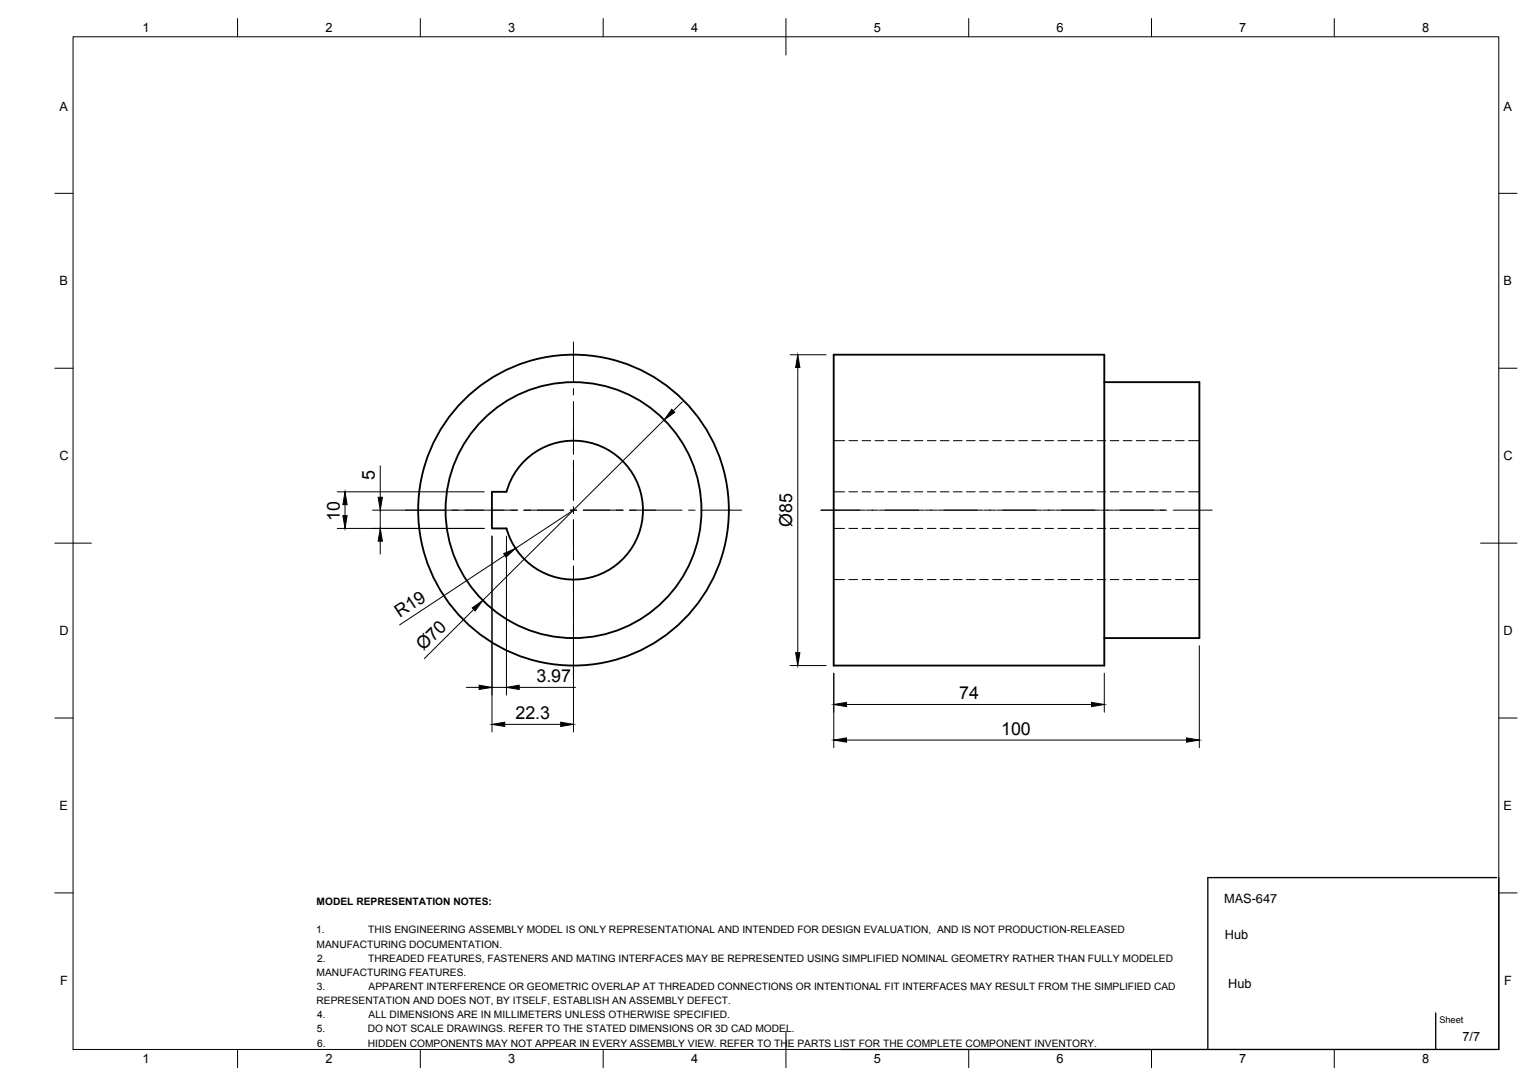
ISO-10303-21;
HEADER;
FILE_DESCRIPTION((''),'2;1');
FILE_NAME('Hub.step','2026-10-09T11:36:02-07:00',(''),(''),'','','');
FILE_SCHEMA (('AUTOMOTIVE_DESIGN { 1 0 10303 214 3 1 1 }'));
ENDSEC;
DATA;
#10=MECHANICAL_DESIGN_GEOMETRIC_PRESENTATION_REPRESENTATION('',(#85),#1549);
#75=SHAPE_REPRESENTATION_RELATIONSHIP('SRR','None',#1584,#80) ;
#80=ADVANCED_BREP_SHAPE_REPRESENTATION('',(#90),#1547) ;
#85=STYLED_ITEM('',(#1615),#90) ;
#90=MANIFOLD_SOLID_BREP('Body1',#847) ;
#120=FACE_BOUND('',#246,.T.) ;
#121=FACE_BOUND('',#248,.T.) ;
#122=FACE_BOUND('',#250,.T.) ;
#127=PLANE('',#988) ;
#128=PLANE('',#989) ;
#129=PLANE('',#990) ;
#130=PLANE('',#991) ;
#131=PLANE('',#992) ;
#132=PLANE('',#993) ;
#168=FACE_OUTER_BOUND('',#242,.T.) ;
#169=FACE_OUTER_BOUND('',#243,.T.) ;
#170=FACE_OUTER_BOUND('',#244,.T.) ;
#171=FACE_OUTER_BOUND('',#245,.T.) ;
#172=FACE_OUTER_BOUND('',#247,.T.) ;
#173=FACE_OUTER_BOUND('',#249,.T.) ;
#174=FACE_OUTER_BOUND('',#251,.T.) ;
#175=FACE_OUTER_BOUND('',#252,.T.) ;
#176=FACE_OUTER_BOUND('',#253,.T.) ;
#242=EDGE_LOOP('',(#699,#700,#701,#702)) ;
#243=EDGE_LOOP('',(#703,#704,#705,#706)) ;
#244=EDGE_LOOP('',(#707,#708,#709,#710)) ;
#245=EDGE_LOOP('',(#711)) ;
#246=EDGE_LOOP('',(#712,#713,#714,#715)) ;
#247=EDGE_LOOP('',(#716)) ;
#248=EDGE_LOOP('',(#717)) ;
#249=EDGE_LOOP('',(#718)) ;
#250=EDGE_LOOP('',(#719,#720,#721,#722)) ;
#251=EDGE_LOOP('',(#723,#724,#725,#726)) ;
#252=EDGE_LOOP('',(#727,#728,#729,#730)) ;
#253=EDGE_LOOP('',(#731,#732,#733,#734)) ;
#284=LINE('',#1444,#332) ;
#285=LINE('',#1450,#333) ;
#286=LINE('',#1457,#334) ;
#287=LINE('',#1460,#335) ;
#288=LINE('',#1464,#336) ;
#289=LINE('',#1465,#337) ;
#290=LINE('',#1466,#338) ;
#291=LINE('',#1470,#339) ;
#292=LINE('',#1472,#340) ;
#293=LINE('',#1473,#341) ;
#294=LINE('',#1475,#342) ;
#295=LINE('',#1477,#343) ;
#332=VECTOR('',#1195,42.5) ;
#333=VECTOR('',#1202,35.) ;
#334=VECTOR('',#1209,1000.) ;
#335=VECTOR('',#1212,1000.) ;
#336=VECTOR('',#1215,1000.) ;
#337=VECTOR('',#1216,1000.) ;
#338=VECTOR('',#1217,1000.) ;
#339=VECTOR('',#1222,1000.) ;
#340=VECTOR('',#1223,1000.) ;
#341=VECTOR('',#1224,1000.) ;
#342=VECTOR('',#1227,1000.) ;
#343=VECTOR('',#1230,1000.) ;
#402=CIRCLE('',#980,42.5) ;
#403=CIRCLE('',#981,42.5) ;
#404=CIRCLE('',#983,35.) ;
#405=CIRCLE('',#984,35.) ;
#406=CIRCLE('',#986,19.) ;
#407=CIRCLE('',#987,19.) ;
#451=VERTEX_POINT('',#1441) ;
#452=VERTEX_POINT('',#1443) ;
#453=VERTEX_POINT('',#1447) ;
#454=VERTEX_POINT('',#1449) ;
#455=VERTEX_POINT('',#1453) ;
#456=VERTEX_POINT('',#1454) ;
#457=VERTEX_POINT('',#1456) ;
#458=VERTEX_POINT('',#1458) ;
#459=VERTEX_POINT('',#1462) ;
#460=VERTEX_POINT('',#1463) ;
#461=VERTEX_POINT('',#1469) ;
#462=VERTEX_POINT('',#1471) ;
#537=EDGE_CURVE('',#451,#451,#402,.T.) ;
#538=EDGE_CURVE('',#451,#452,#284,.T.) ;
#539=EDGE_CURVE('',#452,#452,#403,.T.) ;
#540=EDGE_CURVE('',#453,#453,#404,.T.) ;
#541=EDGE_CURVE('',#453,#454,#285,.T.) ;
#542=EDGE_CURVE('',#454,#454,#405,.T.) ;
#543=EDGE_CURVE('',#455,#456,#406,.T.) ;
#544=EDGE_CURVE('',#457,#455,#286,.T.) ;
#545=EDGE_CURVE('',#457,#458,#407,.T.) ;
#546=EDGE_CURVE('',#458,#456,#287,.T.) ;
#547=EDGE_CURVE('',#459,#460,#288,.T.) ;
#548=EDGE_CURVE('',#460,#458,#289,.T.) ;
#549=EDGE_CURVE('',#457,#459,#290,.T.) ;
#550=EDGE_CURVE('',#461,#456,#291,.T.) ;
#551=EDGE_CURVE('',#462,#461,#292,.T.) ;
#552=EDGE_CURVE('',#455,#462,#293,.T.) ;
#553=EDGE_CURVE('',#460,#461,#294,.T.) ;
#554=EDGE_CURVE('',#459,#462,#295,.T.) ;
#699=ORIENTED_EDGE('',*,*,#537,.F.) ;
#700=ORIENTED_EDGE('',*,*,#538,.T.) ;
#701=ORIENTED_EDGE('',*,*,#539,.T.) ;
#702=ORIENTED_EDGE('',*,*,#538,.F.) ;
#703=ORIENTED_EDGE('',*,*,#540,.F.) ;
#704=ORIENTED_EDGE('',*,*,#541,.T.) ;
#705=ORIENTED_EDGE('',*,*,#542,.T.) ;
#706=ORIENTED_EDGE('',*,*,#541,.F.) ;
#707=ORIENTED_EDGE('',*,*,#543,.F.) ;
#708=ORIENTED_EDGE('',*,*,#544,.F.) ;
#709=ORIENTED_EDGE('',*,*,#545,.T.) ;
#710=ORIENTED_EDGE('',*,*,#546,.T.) ;
#711=ORIENTED_EDGE('',*,*,#540,.T.) ;
#712=ORIENTED_EDGE('',*,*,#547,.T.) ;
#713=ORIENTED_EDGE('',*,*,#548,.T.) ;
#714=ORIENTED_EDGE('',*,*,#545,.F.) ;
#715=ORIENTED_EDGE('',*,*,#549,.T.) ;
#716=ORIENTED_EDGE('',*,*,#537,.T.) ;
#717=ORIENTED_EDGE('',*,*,#542,.F.) ;
#718=ORIENTED_EDGE('',*,*,#539,.F.) ;
#719=ORIENTED_EDGE('',*,*,#543,.T.) ;
#720=ORIENTED_EDGE('',*,*,#550,.F.) ;
#721=ORIENTED_EDGE('',*,*,#551,.F.) ;
#722=ORIENTED_EDGE('',*,*,#552,.F.) ;
#723=ORIENTED_EDGE('',*,*,#550,.T.) ;
#724=ORIENTED_EDGE('',*,*,#546,.F.) ;
#725=ORIENTED_EDGE('',*,*,#548,.F.) ;
#726=ORIENTED_EDGE('',*,*,#553,.T.) ;
#727=ORIENTED_EDGE('',*,*,#551,.T.) ;
#728=ORIENTED_EDGE('',*,*,#553,.F.) ;
#729=ORIENTED_EDGE('',*,*,#547,.F.) ;
#730=ORIENTED_EDGE('',*,*,#554,.T.) ;
#731=ORIENTED_EDGE('',*,*,#552,.T.) ;
#732=ORIENTED_EDGE('',*,*,#554,.F.) ;
#733=ORIENTED_EDGE('',*,*,#549,.F.) ;
#734=ORIENTED_EDGE('',*,*,#544,.T.) ;
#793=CYLINDRICAL_SURFACE('',#979,42.5) ;
#794=CYLINDRICAL_SURFACE('',#982,35.) ;
#795=CYLINDRICAL_SURFACE('',#985,19.) ;
#825=ADVANCED_FACE('',(#168),#793,.T.) ;
#826=ADVANCED_FACE('',(#169),#794,.T.) ;
#827=ADVANCED_FACE('',(#170),#795,.F.) ;
#828=ADVANCED_FACE('',(#171,#120),#127,.F.) ;
#829=ADVANCED_FACE('',(#172,#121),#128,.F.) ;
#830=ADVANCED_FACE('',(#173,#122),#129,.F.) ;
#831=ADVANCED_FACE('',(#174),#130,.F.) ;
#832=ADVANCED_FACE('',(#175),#131,.F.) ;
#833=ADVANCED_FACE('',(#176),#132,.F.) ;
#847=CLOSED_SHELL('',(#825,#826,#827,#828,#829,#830,#831,#832,#833)) ;
#978=AXIS2_PLACEMENT_3D('',#1439,#1189,#1190) ;
#979=AXIS2_PLACEMENT_3D('',#1440,#1191,#1192) ;
#980=AXIS2_PLACEMENT_3D('',#1442,#1193,#1194) ;
#981=AXIS2_PLACEMENT_3D('',#1445,#1196,#1197) ;
#982=AXIS2_PLACEMENT_3D('',#1446,#1198,#1199) ;
#983=AXIS2_PLACEMENT_3D('',#1448,#1200,#1201) ;
#984=AXIS2_PLACEMENT_3D('',#1451,#1203,#1204) ;
#985=AXIS2_PLACEMENT_3D('',#1452,#1205,#1206) ;
#986=AXIS2_PLACEMENT_3D('',#1455,#1207,#1208) ;
#987=AXIS2_PLACEMENT_3D('',#1459,#1210,#1211) ;
#988=AXIS2_PLACEMENT_3D('',#1461,#1213,#1214) ;
#989=AXIS2_PLACEMENT_3D('',#1467,#1218,#1219) ;
#990=AXIS2_PLACEMENT_3D('',#1468,#1220,#1221) ;
#991=AXIS2_PLACEMENT_3D('',#1474,#1225,#1226) ;
#992=AXIS2_PLACEMENT_3D('',#1476,#1228,#1229) ;
#993=AXIS2_PLACEMENT_3D('',#1478,#1231,#1232) ;
#1189=DIRECTION('axis',(0.,0.,1.)) ;
#1190=DIRECTION('refdir',(1.,0.,0.)) ;
#1191=DIRECTION('center_axis',(-1.,0.,0.)) ;
#1192=DIRECTION('ref_axis',(0.,0.,1.)) ;
#1193=DIRECTION('center_axis',(-1.,0.,0.)) ;
#1194=DIRECTION('ref_axis',(0.,0.,1.)) ;
#1195=DIRECTION('',(1.,0.,0.)) ;
#1196=DIRECTION('center_axis',(-1.,0.,0.)) ;
#1197=DIRECTION('ref_axis',(0.,0.,1.)) ;
#1198=DIRECTION('center_axis',(-1.,0.,0.)) ;
#1199=DIRECTION('ref_axis',(0.,0.,1.)) ;
#1200=DIRECTION('center_axis',(-1.,0.,0.)) ;
#1201=DIRECTION('ref_axis',(0.,0.,1.)) ;
#1202=DIRECTION('',(1.,0.,0.)) ;
#1203=DIRECTION('center_axis',(-1.,0.,0.)) ;
#1204=DIRECTION('ref_axis',(0.,0.,1.)) ;
#1205=DIRECTION('center_axis',(-1.,0.,0.)) ;
#1206=DIRECTION('ref_axis',(0.,-1.,-1.83697019872103E-16)) ;
#1207=DIRECTION('center_axis',(-1.,0.,0.)) ;
#1208=DIRECTION('ref_axis',(0.,0.,1.)) ;
#1209=DIRECTION('',(1.,0.,0.)) ;
#1210=DIRECTION('center_axis',(-1.,0.,0.)) ;
#1211=DIRECTION('ref_axis',(0.,0.,1.)) ;
#1212=DIRECTION('',(1.,0.,0.)) ;
#1213=DIRECTION('center_axis',(1.,0.,0.)) ;
#1214=DIRECTION('ref_axis',(0.,0.,-1.)) ;
#1215=DIRECTION('',(0.,0.,1.)) ;
#1216=DIRECTION('',(0.,-1.,0.)) ;
#1217=DIRECTION('',(0.,1.,2.18495691202819E-16)) ;
#1218=DIRECTION('center_axis',(1.,0.,0.)) ;
#1219=DIRECTION('ref_axis',(0.,0.,-1.)) ;
#1220=DIRECTION('center_axis',(-1.,0.,0.)) ;
#1221=DIRECTION('ref_axis',(0.,0.,1.)) ;
#1222=DIRECTION('',(0.,-1.,0.)) ;
#1223=DIRECTION('',(0.,0.,1.)) ;
#1224=DIRECTION('',(0.,1.,2.18495691202819E-16)) ;
#1225=DIRECTION('center_axis',(0.,0.,1.)) ;
#1226=DIRECTION('ref_axis',(1.,0.,0.)) ;
#1227=DIRECTION('',(1.,0.,0.)) ;
#1228=DIRECTION('center_axis',(0.,1.,0.)) ;
#1229=DIRECTION('ref_axis',(0.,0.,1.)) ;
#1230=DIRECTION('',(1.,0.,0.)) ;
#1231=DIRECTION('center_axis',(0.,2.18495691202819E-16,-1.)) ;
#1232=DIRECTION('ref_axis',(0.,1.,2.18495691202819E-16)) ;
#1439=CARTESIAN_POINT('',(0.,0.,0.)) ;
#1440=CARTESIAN_POINT('Origin',(0.,0.,0.)) ;
#1441=CARTESIAN_POINT('',(26.,-5.20474889637625E-15,-42.5)) ;
#1442=CARTESIAN_POINT('Origin',(26.,0.,0.)) ;
#1443=CARTESIAN_POINT('',(100.,-5.20474889637625E-15,-42.5)) ;
#1444=CARTESIAN_POINT('',(0.,-5.20474889637625E-15,-42.5)) ;
#1445=CARTESIAN_POINT('Origin',(100.,0.,0.)) ;
#1446=CARTESIAN_POINT('Origin',(0.,0.,0.)) ;
#1447=CARTESIAN_POINT('',(0.,-4.28626379701574E-15,-35.)) ;
#1448=CARTESIAN_POINT('Origin',(0.,0.,0.)) ;
#1449=CARTESIAN_POINT('',(26.,-4.28626379701574E-15,-35.)) ;
#1450=CARTESIAN_POINT('',(0.,-4.28626379701574E-15,-35.)) ;
#1451=CARTESIAN_POINT('Origin',(26.,0.,0.)) ;
#1452=CARTESIAN_POINT('Origin',(0.,0.,0.)) ;
#1453=CARTESIAN_POINT('',(100.,18.3303027798234,-5.)) ;
#1454=CARTESIAN_POINT('',(100.,18.3303027798234,5.)) ;
#1455=CARTESIAN_POINT('Origin',(100.,0.,0.)) ;
#1456=CARTESIAN_POINT('',(0.,18.3303027798234,-5.)) ;
#1457=CARTESIAN_POINT('',(0.,18.3303027798234,-5.)) ;
#1458=CARTESIAN_POINT('',(0.,18.3303027798234,5.)) ;
#1459=CARTESIAN_POINT('Origin',(0.,0.,0.)) ;
#1460=CARTESIAN_POINT('',(0.,18.3303027798234,5.)) ;
#1461=CARTESIAN_POINT('Origin',(0.,19.,0.)) ;
#1462=CARTESIAN_POINT('',(0.,22.3,-5.)) ;
#1463=CARTESIAN_POINT('',(0.,22.3,5.)) ;
#1464=CARTESIAN_POINT('',(0.,22.3,5.)) ;
#1465=CARTESIAN_POINT('',(0.,22.3,5.)) ;
#1466=CARTESIAN_POINT('',(0.,22.3,-5.)) ;
#1467=CARTESIAN_POINT('Origin',(26.,35.,0.)) ;
#1468=CARTESIAN_POINT('Origin',(100.,42.5,0.)) ;
#1469=CARTESIAN_POINT('',(100.,22.3,5.)) ;
#1470=CARTESIAN_POINT('',(100.,22.3,5.)) ;
#1471=CARTESIAN_POINT('',(100.,22.3,-5.)) ;
#1472=CARTESIAN_POINT('',(100.,22.3,5.)) ;
#1473=CARTESIAN_POINT('',(100.,22.3,-5.)) ;
#1474=CARTESIAN_POINT('Origin',(0.,22.3,5.)) ;
#1475=CARTESIAN_POINT('',(0.,22.3,5.)) ;
#1476=CARTESIAN_POINT('Origin',(0.,22.3,5.)) ;
#1477=CARTESIAN_POINT('',(0.,22.3,-5.)) ;
#1478=CARTESIAN_POINT('Origin',(0.,22.3,-5.)) ;
#1540=UNCERTAINTY_MEASURE_WITH_UNIT(LENGTH_MEASURE(0.01),#1550,
'DISTANCE_ACCURACY_VALUE',
'Maximum model space distance between geometric entities at asserted c
onnectivities') ;
#1542=UNCERTAINTY_MEASURE_WITH_UNIT(LENGTH_MEASURE(0.01),#1550,
'DISTANCE_ACCURACY_VALUE',
'Maximum model space distance between geometric entities at asserted c
onnectivities') ;
#1547=(
GEOMETRIC_REPRESENTATION_CONTEXT(3)
GLOBAL_UNCERTAINTY_ASSIGNED_CONTEXT((#1540))
GLOBAL_UNIT_ASSIGNED_CONTEXT((#1550,#1552,#1553))
REPRESENTATION_CONTEXT('','3D')
) ;
#1549=(
GEOMETRIC_REPRESENTATION_CONTEXT(3)
GLOBAL_UNCERTAINTY_ASSIGNED_CONTEXT((#1542))
GLOBAL_UNIT_ASSIGNED_CONTEXT((#1550,#1552,#1553))
REPRESENTATION_CONTEXT('','3D')
) ;
#1550=(
LENGTH_UNIT()
NAMED_UNIT(*)
SI_UNIT(.MILLI.,.METRE.)
) ;
#1552=(
NAMED_UNIT(*)
PLANE_ANGLE_UNIT()
SI_UNIT($,.RADIAN.)
) ;
#1553=(
NAMED_UNIT(*)
SI_UNIT($,.STERADIAN.)
SOLID_ANGLE_UNIT()
) ;
#1558=SHAPE_DEFINITION_REPRESENTATION(#1564,#1584) ;
#1564=PRODUCT_DEFINITION_SHAPE('',$,#1591) ;
#1584=SHAPE_REPRESENTATION('',(#978),#1547) ;
#1586=PRODUCT_DEFINITION_CONTEXT('part definition',#1606,'design') ;
#1591=PRODUCT_DEFINITION('Hub','Hub',#1597,#1586) ;
#1597=PRODUCT_DEFINITION_FORMATION('',$,#1612) ;
#1606=APPLICATION_CONTEXT(
'Core Data for Automotive Mechanical Design Process') ;
#1607=PRODUCT_CONTEXT('part definition',#1606,'mechanical') ;
#1612=PRODUCT('Hub','Hub',$,(#1607)) ;
#1615=PRESENTATION_STYLE_ASSIGNMENT((#1617)) ;
#1617=SURFACE_STYLE_USAGE(.BOTH.,#1619) ;
#1619=SURFACE_SIDE_STYLE('',(#1621)) ;
#1621=SURFACE_STYLE_FILL_AREA(#1623) ;
#1623=FILL_AREA_STYLE('Opaque(202,209,238)',(#1625)) ;
#1625=FILL_AREA_STYLE_COLOUR('Opaque(202,209,238)',#1627) ;
#1627=COLOUR_RGB('Opaque(202,209,238)', 0.09019608, 0.27058824, 0.51372549) ;
ENDSEC;
END-ISO-10303-21;
